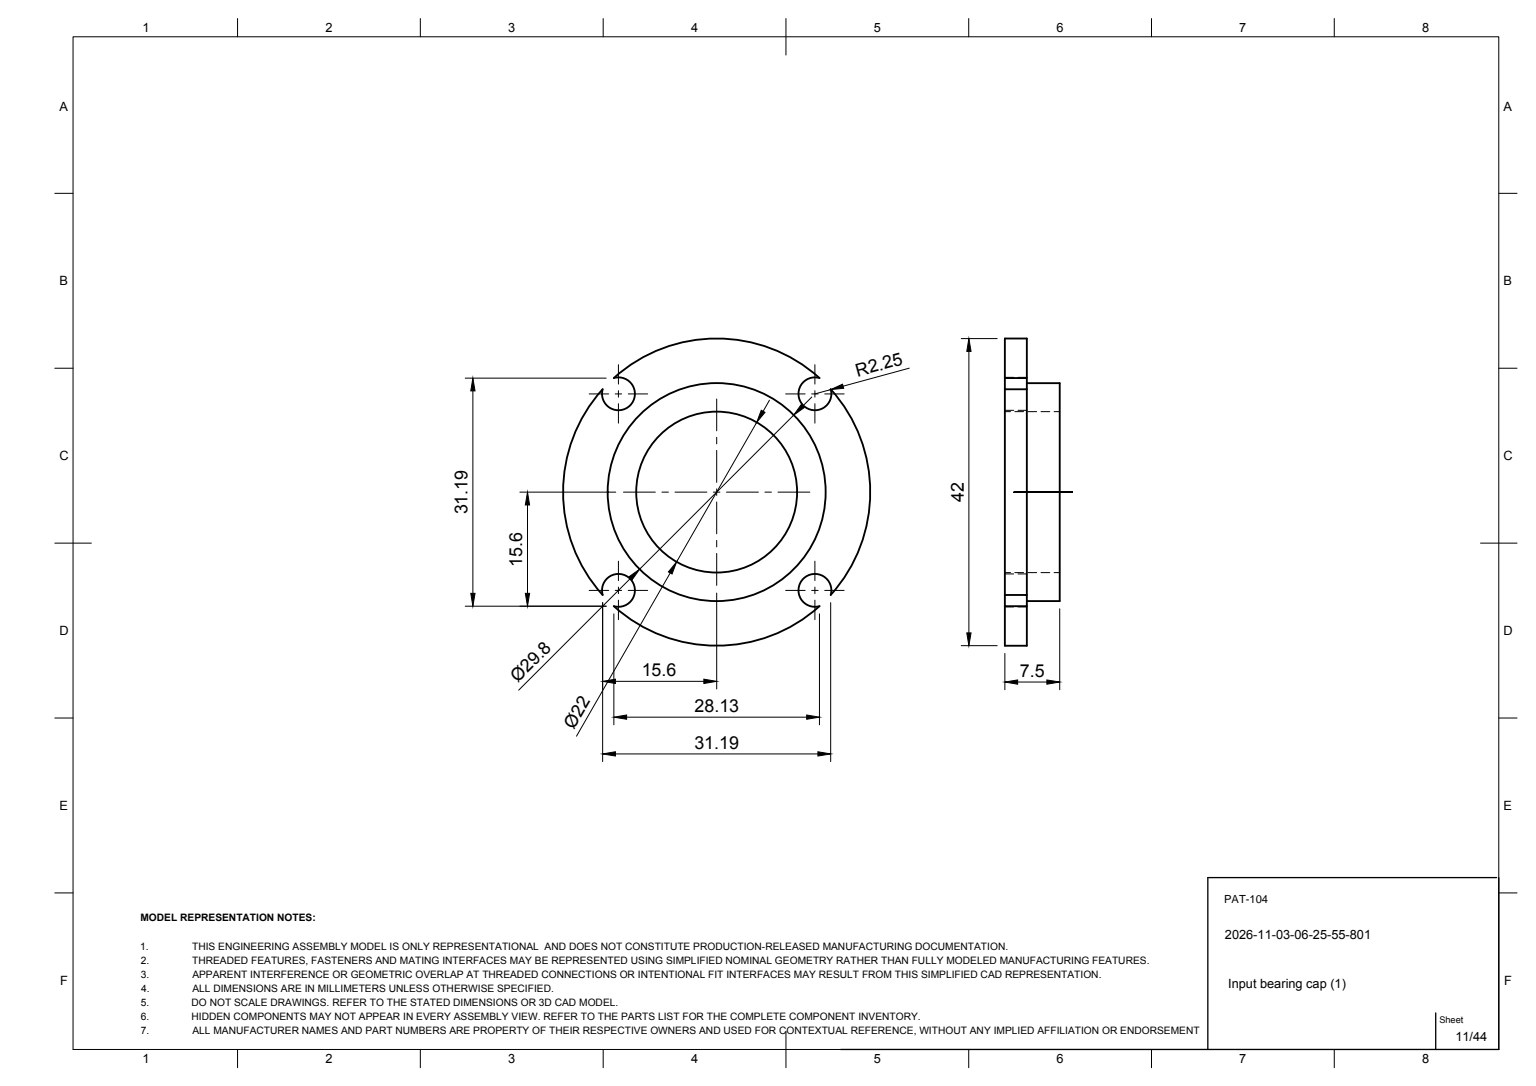
ISO-10303-21;
HEADER;
/* Generated by software containing ST-Developer
 * from STEP Tools, Inc. (www.steptools.com) 
 */

FILE_DESCRIPTION(
/* description */ ('Timing belt drive module 2 mm Pitch Timing 20T-40T'),

/* implementation_level */ '2;1');

FILE_NAME(
/* name */ 'Input bearing cap (1).step',
/* time_stamp */ '2026-10-28T03:25:12-07:00',
/* author */ (''),
/* organization */ (''),
/* preprocessor_version */ 'ST-DEVELOPER v20.2',
/* originating_system */ 'Autodesk Translation Framework v15.17.0.0',
/* authorisation */ '');

FILE_SCHEMA (('AUTOMOTIVE_DESIGN { 1 0 10303 214 3 1 1 }'));
ENDSEC;

DATA;
#10=MECHANICAL_DESIGN_GEOMETRIC_PRESENTATION_REPRESENTATION('',(#530),#17830);
#444=SHAPE_REPRESENTATION_RELATIONSHIP('SRR','None',#18014,#487);
#487=ADVANCED_BREP_SHAPE_REPRESENTATION('',(#588),#17789);
#530=STYLED_ITEM('',(#18317),#588);
#588=MANIFOLD_SOLID_BREP('Body1',#8987);
#670=FACE_BOUND('',#1599,.T.);
#671=FACE_BOUND('',#1606,.T.);
#672=FACE_BOUND('',#1609,.T.);
#818=PLANE('',#9685);
#819=PLANE('',#9701);
#820=PLANE('',#9705);
#1040=FACE_OUTER_BOUND('',#1594,.T.);
#1041=FACE_OUTER_BOUND('',#1595,.T.);
#1042=FACE_OUTER_BOUND('',#1596,.T.);
#1043=FACE_OUTER_BOUND('',#1597,.T.);
#1044=FACE_OUTER_BOUND('',#1598,.T.);
#1045=FACE_OUTER_BOUND('',#1600,.T.);
#1046=FACE_OUTER_BOUND('',#1601,.T.);
#1047=FACE_OUTER_BOUND('',#1602,.T.);
#1048=FACE_OUTER_BOUND('',#1603,.T.);
#1049=FACE_OUTER_BOUND('',#1604,.T.);
#1050=FACE_OUTER_BOUND('',#1605,.T.);
#1051=FACE_OUTER_BOUND('',#1607,.T.);
#1052=FACE_OUTER_BOUND('',#1608,.T.);
#1594=EDGE_LOOP('',(#6151,#6152,#6153,#6154));
#1595=EDGE_LOOP('',(#6155,#6156,#6157,#6158));
#1596=EDGE_LOOP('',(#6159,#6160,#6161,#6162));
#1597=EDGE_LOOP('',(#6163,#6164,#6165,#6166));
#1598=EDGE_LOOP('',(#6167,#6168,#6169,#6170,#6171,#6172,#6173,#6174));
#1599=EDGE_LOOP('',(#6175));
#1600=EDGE_LOOP('',(#6176,#6177,#6178,#6179));
#1601=EDGE_LOOP('',(#6180,#6181,#6182,#6183));
#1602=EDGE_LOOP('',(#6184,#6185,#6186,#6187));
#1603=EDGE_LOOP('',(#6188,#6189,#6190,#6191));
#1604=EDGE_LOOP('',(#6192,#6193,#6194,#6195));
#1605=EDGE_LOOP('',(#6196));
#1606=EDGE_LOOP('',(#6197));
#1607=EDGE_LOOP('',(#6198,#6199,#6200,#6201));
#1608=EDGE_LOOP('',(#6202,#6203,#6204,#6205,#6206,#6207,#6208,#6209));
#1609=EDGE_LOOP('',(#6210));
#2210=CIRCLE('',#9674,0.225);
#2211=CIRCLE('',#9675,0.225);
#2212=CIRCLE('',#9677,0.225);
#2213=CIRCLE('',#9678,0.225);
#2214=CIRCLE('',#9680,0.225);
#2215=CIRCLE('',#9681,0.225);
#2216=CIRCLE('',#9683,0.225);
#2217=CIRCLE('',#9684,0.225);
#2218=CIRCLE('',#9686,2.1);
#2219=CIRCLE('',#9687,2.1);
#2220=CIRCLE('',#9688,2.1);
#2221=CIRCLE('',#9689,2.1);
#2222=CIRCLE('',#9690,1.49);
#2223=CIRCLE('',#9692,2.1);
#2224=CIRCLE('',#9694,2.1);
#2225=CIRCLE('',#9696,2.1);
#2226=CIRCLE('',#9698,2.1);
#2227=CIRCLE('',#9700,1.49);
#2228=CIRCLE('',#9702,1.1);
#2229=CIRCLE('',#9704,1.1);
#2909=LINE('',#14278,#3387);
#2910=LINE('',#14282,#3388);
#2911=LINE('',#14287,#3389);
#2912=LINE('',#14291,#3390);
#2913=LINE('',#14296,#3391);
#2914=LINE('',#14300,#3392);
#2915=LINE('',#14305,#3393);
#2916=LINE('',#14309,#3394);
#2917=LINE('',#14328,#3395);
#2918=LINE('',#14336,#3396);
#3387=VECTOR('',#11244,1.);
#3388=VECTOR('',#11247,1.);
#3389=VECTOR('',#11252,1.);
#3390=VECTOR('',#11255,1.);
#3391=VECTOR('',#11260,1.);
#3392=VECTOR('',#11263,1.);
#3393=VECTOR('',#11268,1.);
#3394=VECTOR('',#11271,1.);
#3395=VECTOR('',#11304,1.49);
#3396=VECTOR('',#11315,1.1);
#3872=VERTEX_POINT('',#14276);
#3873=VERTEX_POINT('',#14277);
#3874=VERTEX_POINT('',#14279);
#3875=VERTEX_POINT('',#14281);
#3876=VERTEX_POINT('',#14285);
#3877=VERTEX_POINT('',#14286);
#3878=VERTEX_POINT('',#14288);
#3879=VERTEX_POINT('',#14290);
#3880=VERTEX_POINT('',#14294);
#3881=VERTEX_POINT('',#14295);
#3882=VERTEX_POINT('',#14297);
#3883=VERTEX_POINT('',#14299);
#3884=VERTEX_POINT('',#14303);
#3885=VERTEX_POINT('',#14304);
#3886=VERTEX_POINT('',#14306);
#3887=VERTEX_POINT('',#14308);
#3888=VERTEX_POINT('',#14316);
#3889=VERTEX_POINT('',#14327);
#3890=VERTEX_POINT('',#14331);
#3891=VERTEX_POINT('',#14334);
#4758=EDGE_CURVE('',#3872,#3873,#2909,.T.);
#4759=EDGE_CURVE('',#3874,#3872,#2210,.T.);
#4760=EDGE_CURVE('',#3875,#3874,#2910,.T.);
#4761=EDGE_CURVE('',#3873,#3875,#2211,.T.);
#4762=EDGE_CURVE('',#3876,#3877,#2911,.T.);
#4763=EDGE_CURVE('',#3878,#3876,#2212,.T.);
#4764=EDGE_CURVE('',#3879,#3878,#2912,.T.);
#4765=EDGE_CURVE('',#3877,#3879,#2213,.T.);
#4766=EDGE_CURVE('',#3880,#3881,#2913,.T.);
#4767=EDGE_CURVE('',#3882,#3880,#2214,.T.);
#4768=EDGE_CURVE('',#3883,#3882,#2914,.T.);
#4769=EDGE_CURVE('',#3881,#3883,#2215,.T.);
#4770=EDGE_CURVE('',#3884,#3885,#2915,.T.);
#4771=EDGE_CURVE('',#3886,#3884,#2216,.T.);
#4772=EDGE_CURVE('',#3887,#3886,#2916,.T.);
#4773=EDGE_CURVE('',#3885,#3887,#2217,.T.);
#4774=EDGE_CURVE('',#3886,#3872,#2218,.T.);
#4775=EDGE_CURVE('',#3882,#3884,#2219,.T.);
#4776=EDGE_CURVE('',#3878,#3880,#2220,.T.);
#4777=EDGE_CURVE('',#3874,#3876,#2221,.T.);
#4778=EDGE_CURVE('',#3888,#3888,#2222,.T.);
#4779=EDGE_CURVE('',#3883,#3885,#2223,.T.);
#4780=EDGE_CURVE('',#3879,#3881,#2224,.T.);
#4781=EDGE_CURVE('',#3887,#3873,#2225,.T.);
#4782=EDGE_CURVE('',#3875,#3877,#2226,.T.);
#4783=EDGE_CURVE('',#3888,#3889,#2917,.T.);
#4784=EDGE_CURVE('',#3889,#3889,#2227,.T.);
#4785=EDGE_CURVE('',#3890,#3890,#2228,.T.);
#4786=EDGE_CURVE('',#3891,#3891,#2229,.T.);
#4787=EDGE_CURVE('',#3891,#3890,#2918,.T.);
#6151=ORIENTED_EDGE('',*,*,#4758,.F.);
#6152=ORIENTED_EDGE('',*,*,#4759,.F.);
#6153=ORIENTED_EDGE('',*,*,#4760,.F.);
#6154=ORIENTED_EDGE('',*,*,#4761,.F.);
#6155=ORIENTED_EDGE('',*,*,#4762,.F.);
#6156=ORIENTED_EDGE('',*,*,#4763,.F.);
#6157=ORIENTED_EDGE('',*,*,#4764,.F.);
#6158=ORIENTED_EDGE('',*,*,#4765,.F.);
#6159=ORIENTED_EDGE('',*,*,#4766,.F.);
#6160=ORIENTED_EDGE('',*,*,#4767,.F.);
#6161=ORIENTED_EDGE('',*,*,#4768,.F.);
#6162=ORIENTED_EDGE('',*,*,#4769,.F.);
#6163=ORIENTED_EDGE('',*,*,#4770,.F.);
#6164=ORIENTED_EDGE('',*,*,#4771,.F.);
#6165=ORIENTED_EDGE('',*,*,#4772,.F.);
#6166=ORIENTED_EDGE('',*,*,#4773,.F.);
#6167=ORIENTED_EDGE('',*,*,#4759,.T.);
#6168=ORIENTED_EDGE('',*,*,#4774,.F.);
#6169=ORIENTED_EDGE('',*,*,#4771,.T.);
#6170=ORIENTED_EDGE('',*,*,#4775,.F.);
#6171=ORIENTED_EDGE('',*,*,#4767,.T.);
#6172=ORIENTED_EDGE('',*,*,#4776,.F.);
#6173=ORIENTED_EDGE('',*,*,#4763,.T.);
#6174=ORIENTED_EDGE('',*,*,#4777,.F.);
#6175=ORIENTED_EDGE('',*,*,#4778,.T.);
#6176=ORIENTED_EDGE('',*,*,#4768,.T.);
#6177=ORIENTED_EDGE('',*,*,#4775,.T.);
#6178=ORIENTED_EDGE('',*,*,#4770,.T.);
#6179=ORIENTED_EDGE('',*,*,#4779,.F.);
#6180=ORIENTED_EDGE('',*,*,#4764,.T.);
#6181=ORIENTED_EDGE('',*,*,#4776,.T.);
#6182=ORIENTED_EDGE('',*,*,#4766,.T.);
#6183=ORIENTED_EDGE('',*,*,#4780,.F.);
#6184=ORIENTED_EDGE('',*,*,#4758,.T.);
#6185=ORIENTED_EDGE('',*,*,#4781,.F.);
#6186=ORIENTED_EDGE('',*,*,#4772,.T.);
#6187=ORIENTED_EDGE('',*,*,#4774,.T.);
#6188=ORIENTED_EDGE('',*,*,#4760,.T.);
#6189=ORIENTED_EDGE('',*,*,#4777,.T.);
#6190=ORIENTED_EDGE('',*,*,#4762,.T.);
#6191=ORIENTED_EDGE('',*,*,#4782,.F.);
#6192=ORIENTED_EDGE('',*,*,#4778,.F.);
#6193=ORIENTED_EDGE('',*,*,#4783,.T.);
#6194=ORIENTED_EDGE('',*,*,#4784,.T.);
#6195=ORIENTED_EDGE('',*,*,#4783,.F.);
#6196=ORIENTED_EDGE('',*,*,#4784,.F.);
#6197=ORIENTED_EDGE('',*,*,#4785,.F.);
#6198=ORIENTED_EDGE('',*,*,#4786,.F.);
#6199=ORIENTED_EDGE('',*,*,#4787,.T.);
#6200=ORIENTED_EDGE('',*,*,#4785,.T.);
#6201=ORIENTED_EDGE('',*,*,#4787,.F.);
#6202=ORIENTED_EDGE('',*,*,#4761,.T.);
#6203=ORIENTED_EDGE('',*,*,#4782,.T.);
#6204=ORIENTED_EDGE('',*,*,#4765,.T.);
#6205=ORIENTED_EDGE('',*,*,#4780,.T.);
#6206=ORIENTED_EDGE('',*,*,#4769,.T.);
#6207=ORIENTED_EDGE('',*,*,#4779,.T.);
#6208=ORIENTED_EDGE('',*,*,#4773,.T.);
#6209=ORIENTED_EDGE('',*,*,#4781,.T.);
#6210=ORIENTED_EDGE('',*,*,#4786,.T.);
#8214=CYLINDRICAL_SURFACE('',#9673,0.225);
#8215=CYLINDRICAL_SURFACE('',#9676,0.225);
#8216=CYLINDRICAL_SURFACE('',#9679,0.225);
#8217=CYLINDRICAL_SURFACE('',#9682,0.225);
#8218=CYLINDRICAL_SURFACE('',#9691,2.1);
#8219=CYLINDRICAL_SURFACE('',#9693,2.1);
#8220=CYLINDRICAL_SURFACE('',#9695,2.1);
#8221=CYLINDRICAL_SURFACE('',#9697,2.1);
#8222=CYLINDRICAL_SURFACE('',#9699,1.49);
#8223=CYLINDRICAL_SURFACE('',#9703,1.1);
#8538=ADVANCED_FACE('',(#1040),#8214,.F.);
#8539=ADVANCED_FACE('',(#1041),#8215,.F.);
#8540=ADVANCED_FACE('',(#1042),#8216,.F.);
#8541=ADVANCED_FACE('',(#1043),#8217,.F.);
#8542=ADVANCED_FACE('',(#1044,#670),#818,.F.);
#8543=ADVANCED_FACE('',(#1045),#8218,.T.);
#8544=ADVANCED_FACE('',(#1046),#8219,.T.);
#8545=ADVANCED_FACE('',(#1047),#8220,.T.);
#8546=ADVANCED_FACE('',(#1048),#8221,.T.);
#8547=ADVANCED_FACE('',(#1049),#8222,.T.);
#8548=ADVANCED_FACE('',(#1050,#671),#819,.F.);
#8549=ADVANCED_FACE('',(#1051),#8223,.F.);
#8550=ADVANCED_FACE('',(#1052,#672),#820,.T.);
#8987=CLOSED_SHELL('',(#8538,#8539,#8540,#8541,#8542,#8543,#8544,#8545,
#8546,#8547,#8548,#8549,#8550));
#9672=AXIS2_PLACEMENT_3D('',#14274,#11240,#11241);
#9673=AXIS2_PLACEMENT_3D('',#14275,#11242,#11243);
#9674=AXIS2_PLACEMENT_3D('',#14280,#11245,#11246);
#9675=AXIS2_PLACEMENT_3D('',#14283,#11248,#11249);
#9676=AXIS2_PLACEMENT_3D('',#14284,#11250,#11251);
#9677=AXIS2_PLACEMENT_3D('',#14289,#11253,#11254);
#9678=AXIS2_PLACEMENT_3D('',#14292,#11256,#11257);
#9679=AXIS2_PLACEMENT_3D('',#14293,#11258,#11259);
#9680=AXIS2_PLACEMENT_3D('',#14298,#11261,#11262);
#9681=AXIS2_PLACEMENT_3D('',#14301,#11264,#11265);
#9682=AXIS2_PLACEMENT_3D('',#14302,#11266,#11267);
#9683=AXIS2_PLACEMENT_3D('',#14307,#11269,#11270);
#9684=AXIS2_PLACEMENT_3D('',#14310,#11272,#11273);
#9685=AXIS2_PLACEMENT_3D('',#14311,#11274,#11275);
#9686=AXIS2_PLACEMENT_3D('',#14312,#11276,#11277);
#9687=AXIS2_PLACEMENT_3D('',#14313,#11278,#11279);
#9688=AXIS2_PLACEMENT_3D('',#14314,#11280,#11281);
#9689=AXIS2_PLACEMENT_3D('',#14315,#11282,#11283);
#9690=AXIS2_PLACEMENT_3D('',#14317,#11284,#11285);
#9691=AXIS2_PLACEMENT_3D('',#14318,#11286,#11287);
#9692=AXIS2_PLACEMENT_3D('',#14319,#11288,#11289);
#9693=AXIS2_PLACEMENT_3D('',#14320,#11290,#11291);
#9694=AXIS2_PLACEMENT_3D('',#14321,#11292,#11293);
#9695=AXIS2_PLACEMENT_3D('',#14322,#11294,#11295);
#9696=AXIS2_PLACEMENT_3D('',#14323,#11296,#11297);
#9697=AXIS2_PLACEMENT_3D('',#14324,#11298,#11299);
#9698=AXIS2_PLACEMENT_3D('',#14325,#11300,#11301);
#9699=AXIS2_PLACEMENT_3D('',#14326,#11302,#11303);
#9700=AXIS2_PLACEMENT_3D('',#14329,#11305,#11306);
#9701=AXIS2_PLACEMENT_3D('',#14330,#11307,#11308);
#9702=AXIS2_PLACEMENT_3D('',#14332,#11309,#11310);
#9703=AXIS2_PLACEMENT_3D('',#14333,#11311,#11312);
#9704=AXIS2_PLACEMENT_3D('',#14335,#11313,#11314);
#9705=AXIS2_PLACEMENT_3D('',#14337,#11316,#11317);
#11240=DIRECTION('axis',(0.,0.,1.));
#11241=DIRECTION('refdir',(1.,0.,0.));
#11242=DIRECTION('center_axis',(0.,1.,0.));
#11243=DIRECTION('ref_axis',(0.707106781186546,0.,0.707106781186549));
#11244=DIRECTION('',(0.,1.,0.));
#11245=DIRECTION('center_axis',(0.,1.,0.));
#11246=DIRECTION('ref_axis',(1.,0.,0.));
#11247=DIRECTION('',(0.,-1.,0.));
#11248=DIRECTION('center_axis',(0.,-1.,0.));
#11249=DIRECTION('ref_axis',(1.,0.,0.));
#11250=DIRECTION('center_axis',(0.,1.,0.));
#11251=DIRECTION('ref_axis',(0.707106781186547,0.,-0.707106781186548));
#11252=DIRECTION('',(0.,1.,0.));
#11253=DIRECTION('center_axis',(0.,1.,0.));
#11254=DIRECTION('ref_axis',(1.,0.,0.));
#11255=DIRECTION('',(0.,-1.,0.));
#11256=DIRECTION('center_axis',(0.,-1.,0.));
#11257=DIRECTION('ref_axis',(1.,0.,0.));
#11258=DIRECTION('center_axis',(0.,1.,0.));
#11259=DIRECTION('ref_axis',(-0.707106781186552,0.,-0.707106781186543));
#11260=DIRECTION('',(0.,1.,0.));
#11261=DIRECTION('center_axis',(0.,1.,0.));
#11262=DIRECTION('ref_axis',(1.,0.,0.));
#11263=DIRECTION('',(0.,-1.,0.));
#11264=DIRECTION('center_axis',(0.,-1.,0.));
#11265=DIRECTION('ref_axis',(1.,0.,0.));
#11266=DIRECTION('center_axis',(0.,1.,0.));
#11267=DIRECTION('ref_axis',(-0.707106781186546,0.,0.707106781186549));
#11268=DIRECTION('',(0.,1.,0.));
#11269=DIRECTION('center_axis',(0.,1.,0.));
#11270=DIRECTION('ref_axis',(1.,0.,0.));
#11271=DIRECTION('',(0.,-1.,0.));
#11272=DIRECTION('center_axis',(0.,-1.,0.));
#11273=DIRECTION('ref_axis',(1.,0.,0.));
#11274=DIRECTION('center_axis',(0.,1.,0.));
#11275=DIRECTION('ref_axis',(1.,0.,0.));
#11276=DIRECTION('center_axis',(0.,1.,0.));
#11277=DIRECTION('ref_axis',(1.,0.,0.));
#11278=DIRECTION('center_axis',(0.,1.,0.));
#11279=DIRECTION('ref_axis',(1.,0.,0.));
#11280=DIRECTION('center_axis',(0.,1.,0.));
#11281=DIRECTION('ref_axis',(1.,0.,0.));
#11282=DIRECTION('center_axis',(0.,1.,0.));
#11283=DIRECTION('ref_axis',(1.,0.,0.));
#11284=DIRECTION('center_axis',(0.,1.,0.));
#11285=DIRECTION('ref_axis',(1.,0.,0.));
#11286=DIRECTION('center_axis',(0.,1.,0.));
#11287=DIRECTION('ref_axis',(1.,0.,0.));
#11288=DIRECTION('center_axis',(0.,1.,0.));
#11289=DIRECTION('ref_axis',(1.,0.,0.));
#11290=DIRECTION('center_axis',(0.,1.,0.));
#11291=DIRECTION('ref_axis',(1.,0.,0.));
#11292=DIRECTION('center_axis',(0.,1.,0.));
#11293=DIRECTION('ref_axis',(1.,0.,0.));
#11294=DIRECTION('center_axis',(0.,1.,0.));
#11295=DIRECTION('ref_axis',(1.,0.,0.));
#11296=DIRECTION('center_axis',(0.,1.,0.));
#11297=DIRECTION('ref_axis',(1.,0.,0.));
#11298=DIRECTION('center_axis',(0.,1.,0.));
#11299=DIRECTION('ref_axis',(-1.,0.,-1.22464679914735E-16));
#11300=DIRECTION('center_axis',(0.,1.,0.));
#11301=DIRECTION('ref_axis',(1.,0.,0.));
#11302=DIRECTION('center_axis',(0.,1.,0.));
#11303=DIRECTION('ref_axis',(1.,0.,0.));
#11304=DIRECTION('',(0.,-1.,0.));
#11305=DIRECTION('center_axis',(0.,1.,0.));
#11306=DIRECTION('ref_axis',(1.,0.,0.));
#11307=DIRECTION('center_axis',(0.,1.,0.));
#11308=DIRECTION('ref_axis',(1.,0.,0.));
#11309=DIRECTION('center_axis',(0.,-1.,0.));
#11310=DIRECTION('ref_axis',(1.,0.,0.));
#11311=DIRECTION('center_axis',(0.,1.,0.));
#11312=DIRECTION('ref_axis',(1.,0.,0.));
#11313=DIRECTION('center_axis',(0.,-1.,0.));
#11314=DIRECTION('ref_axis',(1.,0.,0.));
#11315=DIRECTION('',(0.,-1.,0.));
#11316=DIRECTION('center_axis',(0.,1.,0.));
#11317=DIRECTION('ref_axis',(1.,0.,0.));
#14274=CARTESIAN_POINT('',(0.,0.,0.));
#14275=CARTESIAN_POINT('Origin',(-1.34350288425444,1.7,5.65649711574556));
#14276=CARTESIAN_POINT('',(-1.40634555589641,1.8,5.4404512904656));
#14277=CARTESIAN_POINT('',(-1.40634555589641,2.1,5.4404512904656));
#14278=CARTESIAN_POINT('',(-1.40634555589641,1.7,5.4404512904656));
#14279=CARTESIAN_POINT('',(-1.5595487095344,1.8,5.59365444410359));
#14280=CARTESIAN_POINT('Origin',(-1.34350288425444,1.8,5.65649711574556));
#14281=CARTESIAN_POINT('',(-1.5595487095344,2.1,5.59365444410359));
#14282=CARTESIAN_POINT('',(-1.5595487095344,1.7,5.59365444410359));
#14283=CARTESIAN_POINT('Origin',(-1.34350288425444,2.1,5.65649711574556));
#14284=CARTESIAN_POINT('Origin',(-1.34350288425444,1.7,8.34350288425444));
#14285=CARTESIAN_POINT('',(-1.5595487095344,1.8,8.40634555589641));
#14286=CARTESIAN_POINT('',(-1.5595487095344,2.1,8.40634555589641));
#14287=CARTESIAN_POINT('',(-1.5595487095344,1.7,8.40634555589641));
#14288=CARTESIAN_POINT('',(-1.40634555589641,1.8,8.5595487095344));
#14289=CARTESIAN_POINT('Origin',(-1.34350288425444,1.8,8.34350288425444));
#14290=CARTESIAN_POINT('',(-1.40634555589641,2.1,8.5595487095344));
#14291=CARTESIAN_POINT('',(-1.40634555589641,1.7,8.5595487095344));
#14292=CARTESIAN_POINT('Origin',(-1.34350288425444,2.1,8.34350288425444));
#14293=CARTESIAN_POINT('Origin',(1.34350288425444,1.7,8.34350288425444));
#14294=CARTESIAN_POINT('',(1.40634555589641,1.8,8.5595487095344));
#14295=CARTESIAN_POINT('',(1.40634555589641,2.1,8.5595487095344));
#14296=CARTESIAN_POINT('',(1.40634555589641,1.7,8.5595487095344));
#14297=CARTESIAN_POINT('',(1.5595487095344,1.8,8.40634555589641));
#14298=CARTESIAN_POINT('Origin',(1.34350288425444,1.8,8.34350288425444));
#14299=CARTESIAN_POINT('',(1.5595487095344,2.1,8.40634555589641));
#14300=CARTESIAN_POINT('',(1.5595487095344,1.7,8.40634555589641));
#14301=CARTESIAN_POINT('Origin',(1.34350288425444,2.1,8.34350288425444));
#14302=CARTESIAN_POINT('Origin',(1.34350288425444,1.7,5.65649711574556));
#14303=CARTESIAN_POINT('',(1.5595487095344,1.8,5.59365444410359));
#14304=CARTESIAN_POINT('',(1.5595487095344,2.1,5.59365444410359));
#14305=CARTESIAN_POINT('',(1.5595487095344,1.7,5.59365444410359));
#14306=CARTESIAN_POINT('',(1.40634555589641,1.8,5.4404512904656));
#14307=CARTESIAN_POINT('Origin',(1.34350288425444,1.8,5.65649711574556));
#14308=CARTESIAN_POINT('',(1.40634555589641,2.1,5.4404512904656));
#14309=CARTESIAN_POINT('',(1.40634555589641,1.7,5.4404512904656));
#14310=CARTESIAN_POINT('Origin',(1.34350288425444,2.1,5.65649711574556));
#14311=CARTESIAN_POINT('Origin',(0.,1.8,7.));
#14312=CARTESIAN_POINT('Origin',(0.,1.8,7.));
#14313=CARTESIAN_POINT('Origin',(0.,1.8,7.));
#14314=CARTESIAN_POINT('Origin',(0.,1.8,7.));
#14315=CARTESIAN_POINT('Origin',(0.,1.8,7.));
#14316=CARTESIAN_POINT('',(-1.49,1.8,7.));
#14317=CARTESIAN_POINT('Origin',(0.,1.8,7.));
#14318=CARTESIAN_POINT('Origin',(0.,1.8,7.));
#14319=CARTESIAN_POINT('Origin',(0.,2.1,7.));
#14320=CARTESIAN_POINT('Origin',(0.,1.8,7.));
#14321=CARTESIAN_POINT('Origin',(0.,2.1,7.));
#14322=CARTESIAN_POINT('Origin',(0.,1.8,7.));
#14323=CARTESIAN_POINT('Origin',(0.,2.1,7.));
#14324=CARTESIAN_POINT('Origin',(0.,1.8,7.));
#14325=CARTESIAN_POINT('Origin',(0.,2.1,7.));
#14326=CARTESIAN_POINT('Origin',(0.,1.35,7.));
#14327=CARTESIAN_POINT('',(-1.49,1.35,7.));
#14328=CARTESIAN_POINT('',(-1.49,1.35,7.));
#14329=CARTESIAN_POINT('Origin',(0.,1.35,7.));
#14330=CARTESIAN_POINT('Origin',(0.,1.35,7.));
#14331=CARTESIAN_POINT('',(-1.1,1.35,7.));
#14332=CARTESIAN_POINT('Origin',(0.,1.35,7.));
#14333=CARTESIAN_POINT('Origin',(0.,1.8,7.));
#14334=CARTESIAN_POINT('',(-1.1,2.1,7.));
#14335=CARTESIAN_POINT('Origin',(0.,2.1,7.));
#14336=CARTESIAN_POINT('',(-1.1,1.8,7.));
#14337=CARTESIAN_POINT('Origin',(0.,2.1,7.));
#17739=UNCERTAINTY_MEASURE_WITH_UNIT(LENGTH_MEASURE(0.001),#17831,
'DISTANCE_ACCURACY_VALUE',
'Maximum model space distance between geometric entities at asserted c
onnectivities');
#17780=UNCERTAINTY_MEASURE_WITH_UNIT(LENGTH_MEASURE(0.001),#17831,
'DISTANCE_ACCURACY_VALUE',
'Maximum model space distance between geometric entities at asserted c
onnectivities');
#17789=(
GEOMETRIC_REPRESENTATION_CONTEXT(3)
GLOBAL_UNCERTAINTY_ASSIGNED_CONTEXT((#17739))
GLOBAL_UNIT_ASSIGNED_CONTEXT((#17831,#17833,#17834))
REPRESENTATION_CONTEXT('','3D')
);
#17830=(
GEOMETRIC_REPRESENTATION_CONTEXT(3)
GLOBAL_UNCERTAINTY_ASSIGNED_CONTEXT((#17780))
GLOBAL_UNIT_ASSIGNED_CONTEXT((#17831,#17833,#17834))
REPRESENTATION_CONTEXT('','3D')
);
#17831=(
LENGTH_UNIT()
NAMED_UNIT(*)
SI_UNIT(.CENTI.,.METRE.)
);
#17833=(
NAMED_UNIT(*)
PLANE_ANGLE_UNIT()
SI_UNIT($,.RADIAN.)
);
#17834=(
NAMED_UNIT(*)
SI_UNIT($,.STERADIAN.)
SOLID_ANGLE_UNIT()
);
#17843=SHAPE_DEFINITION_REPRESENTATION(#17892,#18014);
#17892=PRODUCT_DEFINITION_SHAPE('',$,#18064);
#18014=SHAPE_REPRESENTATION('',(#9672),#17789);
#18055=PRODUCT_DEFINITION_CONTEXT('part definition',#18204,'design');
#18064=PRODUCT_DEFINITION('Input bearing cap (1)','Input bearing cap (1)',
#18113,#18055);
#18113=PRODUCT_DEFINITION_FORMATION('',$,#18214);
#18204=APPLICATION_CONTEXT(
'Core Data for Automotive Mechanical Design Process');
#18205=PRODUCT_CONTEXT('part definition',#18204,'mechanical');
#18214=PRODUCT('Input bearing cap (1)','Input bearing cap (1)',
'Input bearing cap (1)',(#18205));
#18311=COLOUR_RGB('Grey',0.48,0.52,0.57);
#18312=FILL_AREA_STYLE_COLOUR('',#18311);
#18313=FILL_AREA_STYLE('',(#18312));
#18314=SURFACE_STYLE_FILL_AREA(#18313);
#18315=SURFACE_SIDE_STYLE('',(#18314));
#18316=SURFACE_STYLE_USAGE(.BOTH.,#18315);
#18317=PRESENTATION_STYLE_ASSIGNMENT((#18316));
ENDSEC;
END-ISO-10303-21;
